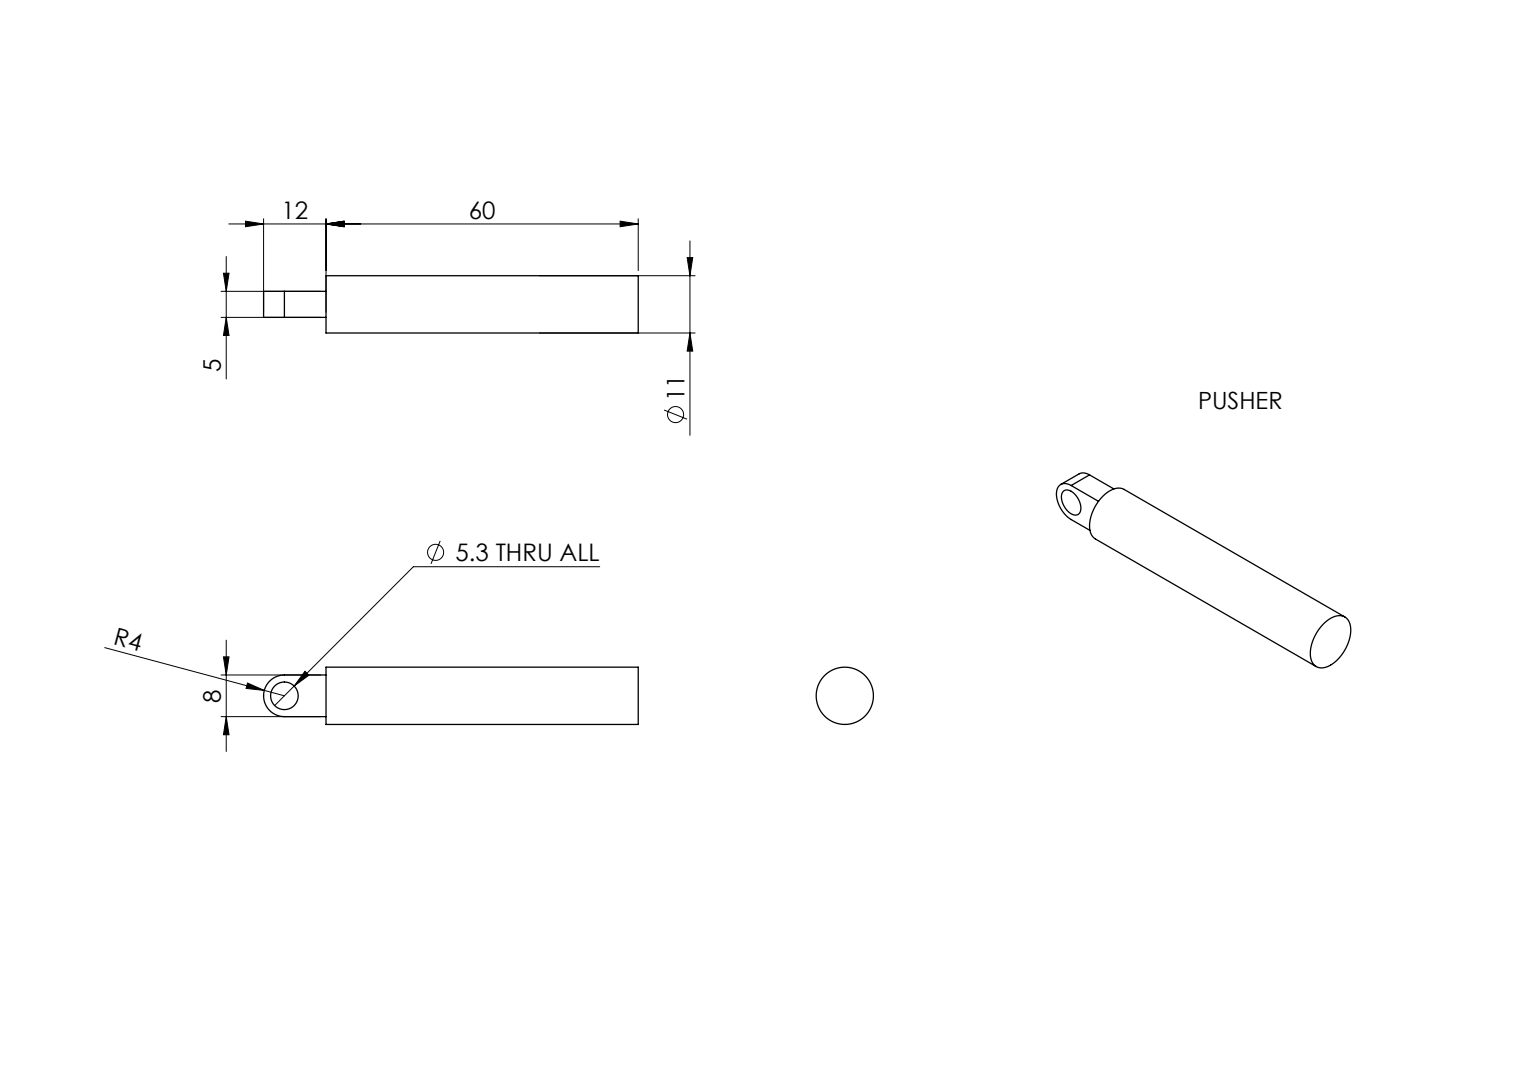
ISO-10303-21;
HEADER;
FILE_DESCRIPTION (('STEP AP214'),
    '1' );
FILE_NAME ('pusher.step',
    '2026-10-31T03:36:27',
    ( '' ),
    ( '' ),
    'SwSTEP 2.0',
    'SolidWorks 2026',
    '' );
FILE_SCHEMA (( 'AUTOMOTIVE_DESIGN' ));
ENDSEC;

DATA;
#89=DIRECTION ( 'NONE',  ( -1.000000000000000000, -6.123233995736766036E-17, 0.000000000000000000 ) ) ;
#381=VECTOR ( 'NONE', #24853, 1000.000000000000000 ) ;
#405=CARTESIAN_POINT ( 'NONE',  ( -69.00000000000002842, 214.0000000000000000, -2.499999999999998668 ) ) ;
#724=AXIS2_PLACEMENT_3D ( 'NONE', #30085, #15119, #33117 ) ;
#815=VERTEX_POINT ( 'NONE', #7521 ) ;
#993=EDGE_LOOP ( 'NONE', ( #26998, #21016, #13480, #17384 ) ) ;
#1044=CARTESIAN_POINT ( 'NONE',  ( -81.00000000000002842, 210.0000000000000000, 2.500000000000001332 ) ) ;
#1193=AXIS2_PLACEMENT_3D ( 'NONE', #20299, #5873, #32024 ) ;
#1362=UNCERTAINTY_MEASURE_WITH_UNIT (LENGTH_MEASURE( 1.000000000000000082E-05 ), #30394, 'distance_accuracy_value', 'NONE');
#1421=ORIENTED_EDGE ( 'NONE', *, *, #25932, .T. ) ;
#1435=DIRECTION ( 'NONE',  ( -1.000000000000000000, -6.123233995736766036E-17, 0.000000000000000000 ) ) ;
#1515=ORIENTED_EDGE ( 'NONE', *, *, #28122, .T. ) ;
#1630=EDGE_CURVE ( 'NONE', #12051, #26056, #3822, .T. ) ;
#1711=CIRCLE ( 'NONE', #36816, 4.000000000000003553 ) ;
#1772=DIRECTION ( 'NONE',  ( 0.000000000000000000, -0.000000000000000000, 1.000000000000000000 ) ) ;
#1802=CARTESIAN_POINT ( 'NONE',  ( -81.00000000000002842, 206.0000000000000000, -2.499999999999998668 ) ) ;
#1831=EDGE_CURVE ( 'NONE', #37491, #32439, #17831, .T. ) ;
#1850=EDGE_LOOP ( 'NONE', ( #28320, #13238, #13654, #30388 ) ) ;
#1911=ORIENTED_EDGE ( 'NONE', *, *, #28122, .F. ) ;
#2035=ORIENTED_EDGE ( 'NONE', *, *, #13992, .T. ) ;
#2126=UNCERTAINTY_MEASURE_WITH_UNIT (LENGTH_MEASURE( 1.000000000000000082E-05 ), #20862, 'distance_accuracy_value', 'NONE');
#2132=PRESENTATION_STYLE_ASSIGNMENT (( #28100 ) ) ;
#2262=VERTEX_POINT ( 'NONE', #29366 ) ;
#2357=VERTEX_POINT ( 'NONE', #405 ) ;
#2450=EDGE_LOOP ( 'NONE', ( #21675, #11995 ) ) ;
#2453=DIRECTION ( 'NONE',  ( -0.000000000000000000, 0.000000000000000000, -1.000000000000000000 ) ) ;
#2550=DIRECTION ( 'NONE',  ( 1.659705900203722642E-32, -2.710505431213758127E-16, -1.000000000000000000 ) ) ;
#2706=CARTESIAN_POINT ( 'NONE',  ( -81.00000000000002842, 206.0000000000000000, 2.500000000000002220 ) ) ;
#2729=CARTESIAN_POINT ( 'NONE',  ( -77.00000000000002842, 210.0000000000000000, -2.499999999999998668 ) ) ;
#2863=EDGE_CURVE ( 'NONE', #23355, #12420, #31331, .T. ) ;
#2931=ORIENTED_EDGE ( 'NONE', *, *, #14124, .T. ) ;
#3005=APPLICATION_CONTEXT ( 'automotive_design' ) ;
#3086=CIRCLE ( 'NONE', #4905, 4.000000000000003553 ) ;
#3101=DIRECTION ( 'NONE',  ( 1.000000000000000000, 6.123233995736766036E-17, -0.000000000000000000 ) ) ;
#3149=CARTESIAN_POINT ( 'NONE',  ( -69.00000000000002842, 210.0000000000000000, 0.000000000000000000 ) ) ;
#3179=ORIENTED_EDGE ( 'NONE', *, *, #27550, .T. ) ;
#3259=CARTESIAN_POINT ( 'NONE',  ( -69.00000000000002842, 206.0000000000000000, 2.500000000000002220 ) ) ;
#3322=ORIENTED_EDGE ( 'NONE', *, *, #16398, .T. ) ;
#3446=ADVANCED_FACE ( 'NONE', ( #16857 ), #11157, .F. ) ;
#3460=CARTESIAN_POINT ( 'NONE',  ( -77.00000000000002842, 206.0000000000000000, 2.500000000000002220 ) ) ;
#3489=FACE_OUTER_BOUND ( 'NONE', #993, .T. ) ;
#3523=EDGE_LOOP ( 'NONE', ( #30051, #36717 ) ) ;
#3627=DIRECTION ( 'NONE',  ( 0.000000000000000000, -1.000000000000000000, 0.000000000000000000 ) ) ;
#3812=EDGE_CURVE ( 'NONE', #27158, #34283, #15876, .T. ) ;
#3822=CIRCLE ( 'NONE', #29851, 2.649999999999999467 ) ;
#3891=AXIS2_PLACEMENT_3D ( 'NONE', #8061, #2550, #6277 ) ;
#4004=DIRECTION ( 'NONE',  ( -0.000000000000000000, -0.000000000000000000, -1.000000000000000000 ) ) ;
#4041=AXIS2_PLACEMENT_3D ( 'NONE', #30951, #17105, #10662 ) ;
#4088=PLANE ( 'NONE',  #11659 ) ;
#4609=DIRECTION ( 'NONE',  ( 1.000000000000000000, 6.123233995736766036E-17, 0.000000000000000000 ) ) ;
#4651=DIRECTION ( 'NONE',  ( 0.000000000000000000, 0.000000000000000000, 1.000000000000000000 ) ) ;
#4762=DIRECTION ( 'NONE',  ( -1.659705900203722642E-32, 2.710505431213758127E-16, 1.000000000000000000 ) ) ;
#4766=ORIENTED_EDGE ( 'NONE', *, *, #18461, .F. ) ;
#4775=CARTESIAN_POINT ( 'NONE',  ( -69.00000000000002842, 206.0000000000000000, -2.499999999999998668 ) ) ;
#4905=AXIS2_PLACEMENT_3D ( 'NONE', #10816, #16142, #10443 ) ;
#4970=CARTESIAN_POINT ( 'NONE',  ( -74.35000000000002274, 210.0000000000000000, 5.000000000000000000 ) ) ;
#4973=SURFACE_STYLE_FILL_AREA ( #36251 ) ;
#4979=PLANE ( 'NONE',  #14973 ) ;
#5010=AXIS2_PLACEMENT_3D ( 'NONE', #7498, #24558, #19074 ) ;
#5293=ORIENTED_EDGE ( 'NONE', *, *, #27550, .F. ) ;
#5521=CYLINDRICAL_SURFACE ( 'NONE', #4041, 5.500000000000005329 ) ;
#5525=CARTESIAN_POINT ( 'NONE',  ( -77.00000000000002842, 214.0000000000000000, -2.499999999999998668 ) ) ;
#5671=CIRCLE ( 'NONE', #6276, 5.500000000000005329 ) ;
#5854=FACE_BOUND ( 'NONE', #17149, .T. ) ;
#5873=DIRECTION ( 'NONE',  ( -1.000000000000000000, -6.123233995736766036E-17, 0.000000000000000000 ) ) ;
#6115=VECTOR ( 'NONE', #25968, 1000.000000000000000 ) ;
#6276=AXIS2_PLACEMENT_3D ( 'NONE', #21708, #24542, #32879 ) ;
#6277=DIRECTION ( 'NONE',  ( 0.000000000000000000, 1.000000000000000000, -3.273063162220408568E-16 ) ) ;
#6300=EDGE_CURVE ( 'NONE', #12051, #34283, #28629, .T. ) ;
#6339=DIRECTION ( 'NONE',  ( -0.000000000000000000, -0.000000000000000000, 1.000000000000000000 ) ) ;
#6347=CARTESIAN_POINT ( 'NONE',  ( -81.00000000000002842, 210.0000000000000000, -2.499999999999998668 ) ) ;
#6359=EDGE_LOOP ( 'NONE', ( #16449, #32660, #37421, #24323 ) ) ;
#6405=EDGE_LOOP ( 'NONE', ( #22858, #25663, #2931, #16829, #11316 ) ) ;
#6528=CARTESIAN_POINT ( 'NONE',  ( -77.00000000000002842, 210.0000000000000000, 5.000000000000000000 ) ) ;
#6534=DIRECTION ( 'NONE',  ( 6.123233995736766036E-17, -1.000000000000000000, 0.000000000000000000 ) ) ;
#6740=DIRECTION ( 'NONE',  ( 0.000000000000000000, 0.000000000000000000, 1.000000000000000000 ) ) ;
#6937=VECTOR ( 'NONE', #24097, 1000.000000000000000 ) ;
#7125=CARTESIAN_POINT ( 'NONE',  ( -77.00000000000002842, 210.0000000000000000, 0.000000000000000000 ) ) ;
#7239=LINE ( 'NONE', #13107, #26015 ) ;
#7292=DIRECTION ( 'NONE',  ( -1.659705900203722642E-32, 2.710505431213758127E-16, 1.000000000000000000 ) ) ;
#7314=DIRECTION ( 'NONE',  ( 1.000000000000000000, 0.000000000000000000, -0.000000000000000000 ) ) ;
#7473=ORIENTED_EDGE ( 'NONE', *, *, #16912, .T. ) ;
#7498=CARTESIAN_POINT ( 'NONE',  ( -9.000000000000024869, 210.0000000000000000, 0.000000000000000000 ) ) ;
#7521=CARTESIAN_POINT ( 'NONE',  ( -77.00000000000002842, 214.0000000000000000, -2.499999999999998668 ) ) ;
#7829=CARTESIAN_POINT ( 'NONE',  ( -81.00000000000002842, 214.0000000000000000, -2.499999999999998668 ) ) ;
#7839=CARTESIAN_POINT ( 'NONE',  ( -81.00000000000002842, 214.0000000000000000, -2.499999999999998668 ) ) ;
#8011=LINE ( 'NONE', #7829, #22826 ) ;
#8061=CARTESIAN_POINT ( 'NONE',  ( -77.00000000000002842, 210.0000000000000000, 2.500000000000001332 ) ) ;
#8248=DIRECTION ( 'NONE',  ( 0.000000000000000000, -0.000000000000000000, 1.000000000000000000 ) ) ;
#8585=DIRECTION ( 'NONE',  ( -1.000000000000000000, -6.123233995736766036E-17, 0.000000000000000000 ) ) ;
#8679=CARTESIAN_POINT ( 'NONE',  ( -77.00000000000002842, 214.0000000000000000, 2.500000000000000000 ) ) ;
#8689=ORIENTED_EDGE ( 'NONE', *, *, #32176, .F. ) ;
#8734=PRODUCT_DEFINITION_FORMATION_WITH_SPECIFIED_SOURCE ( 'ANY', '', #37371, .NOT_KNOWN. ) ;
#8743=DIRECTION ( 'NONE',  ( 1.659705900203722642E-32, -2.710505431213758127E-16, -1.000000000000000000 ) ) ;
#8774=DIRECTION ( 'NONE',  ( -0.000000000000000000, -0.000000000000000000, -1.000000000000000000 ) ) ;
#9133=VECTOR ( 'NONE', #17110, 1000.000000000000000 ) ;
#9159=ORIENTED_EDGE ( 'NONE', *, *, #37039, .F. ) ;
#9224=LINE ( 'NONE', #20990, #13139 ) ;
#9590=AXIS2_PLACEMENT_3D ( 'NONE', #15254, #27183, #6534 ) ;
#9662=( NAMED_UNIT ( * ) PLANE_ANGLE_UNIT ( ) SI_UNIT ( $, .RADIAN. ) );
#9682=ORIENTED_EDGE ( 'NONE', *, *, #36803, .T. ) ;
#9903=AXIS2_PLACEMENT_3D ( 'NONE', #7125, #6740, #18315 ) ;
#9929=DIRECTION ( 'NONE',  ( 1.000000000000000000, 0.000000000000000000, 0.000000000000000000 ) ) ;
#10065=EDGE_CURVE ( 'NONE', #2262, #12420, #12265, .T. ) ;
#10071=EDGE_CURVE ( 'NONE', #2262, #26075, #34298, .T. ) ;
#10173=FACE_OUTER_BOUND ( 'NONE', #6359, .T. ) ;
#10277=ADVANCED_FACE ( 'NONE', ( #5854, #31452 ), #4088, .F. ) ;
#10304=VECTOR ( 'NONE', #30574, 1000.000000000000000 ) ;
#10325=EDGE_CURVE ( 'NONE', #21823, #14348, #30432, .T. ) ;
#10430=DIRECTION ( 'NONE',  ( 1.000000000000000000, 6.123233995736766036E-17, -0.000000000000000000 ) ) ;
#10443=DIRECTION ( 'NONE',  ( 1.000000000000000000, 0.000000000000000000, 0.000000000000000000 ) ) ;
#10487=DIRECTION ( 'NONE',  ( 1.000000000000000000, 0.000000000000000000, 0.000000000000000000 ) ) ;
#10662=DIRECTION ( 'NONE',  ( 0.000000000000000000, -1.000000000000000000, 0.000000000000000000 ) ) ;
#10816=CARTESIAN_POINT ( 'NONE',  ( -77.00000000000002842, 210.0000000000000000, -2.499999999999998668 ) ) ;
#10849=FACE_OUTER_BOUND ( 'NONE', #16526, .T. ) ;
#10916=FACE_OUTER_BOUND ( 'NONE', #18657, .T. ) ;
#10984=ORIENTED_EDGE ( 'NONE', *, *, #10071, .T. ) ;
#11076=AXIS2_PLACEMENT_3D ( 'NONE', #33553, #2453, #16876 ) ;
#11092=STYLED_ITEM ( 'NONE', ( #2132 ), #27327 ) ;
#11157=CYLINDRICAL_SURFACE ( 'NONE', #22531, 2.649999999999999467 ) ;
#11316=ORIENTED_EDGE ( 'NONE', *, *, #25932, .F. ) ;
#11384=CARTESIAN_POINT ( 'NONE',  ( -74.35000000000002274, 210.0000000000000000, -2.499999999999998668 ) ) ;
#11530=VERTEX_POINT ( 'NONE', #8679 ) ;
#11574=DIRECTION ( 'NONE',  ( -0.000000000000000000, -0.000000000000000000, 1.000000000000000000 ) ) ;
#11609=CARTESIAN_POINT ( 'NONE',  ( -81.00000000000002842, 206.0000000000000000, -2.499999999999998668 ) ) ;
#11659=AXIS2_PLACEMENT_3D ( 'NONE', #1802, #30245, #7314 ) ;
#11676=ADVANCED_FACE ( 'NONE', ( #10173 ), #29889, .T. ) ;
#11984=LINE ( 'NONE', #29224, #22400 ) ;
#11995=ORIENTED_EDGE ( 'NONE', *, *, #32176, .T. ) ;
#12051=VERTEX_POINT ( 'NONE', #25137 ) ;
#12152=DIRECTION ( 'NONE',  ( -1.000000000000000000, -6.123233995736766036E-17, 0.000000000000000000 ) ) ;
#12216=ADVANCED_FACE ( 'NONE', ( #10916 ), #34039, .T. ) ;
#12265=CIRCLE ( 'NONE', #11076, 4.000000000000003553 ) ;
#12420=VERTEX_POINT ( 'NONE', #6347 ) ;
#12453=ADVANCED_FACE ( 'NONE', ( #30408, #33247 ), #15631, .T. ) ;
#12533=LINE ( 'NONE', #35453, #6937 ) ;
#12549=CARTESIAN_POINT ( 'NONE',  ( -74.35000000000002274, 210.0000000000000000, 2.500000000000001332 ) ) ;
#12693=APPLICATION_CONTEXT ( 'automotive_design' ) ;
#12839=EDGE_CURVE ( 'NONE', #11530, #23355, #1711, .T. ) ;
#13107=CARTESIAN_POINT ( 'NONE',  ( -77.00000000000002842, 206.0000000000000000, -2.499999999999998668 ) ) ;
#13139=VECTOR ( 'NONE', #1435, 1000.000000000000000 ) ;
#13238=ORIENTED_EDGE ( 'NONE', *, *, #25674, .F. ) ;
#13329=SURFACE_SIDE_STYLE ('',( #4973 ) ) ;
#13480=ORIENTED_EDGE ( 'NONE', *, *, #3812, .F. ) ;
#13510=DIRECTION ( 'NONE',  ( -0.000000000000000000, -0.000000000000000000, 1.000000000000000000 ) ) ;
#13654=ORIENTED_EDGE ( 'NONE', *, *, #28096, .T. ) ;
#13710=( LENGTH_UNIT ( ) NAMED_UNIT ( * ) SI_UNIT ( .MILLI., .METRE. ) );
#13868=CARTESIAN_POINT ( 'NONE',  ( -69.00000000000002842, 206.0000000000000000, -2.499999999999998668 ) ) ;
#13930=ORIENTED_EDGE ( 'NONE', *, *, #25674, .T. ) ;
#13992=EDGE_CURVE ( 'NONE', #14430, #2262, #7239, .T. ) ;
#14004=DIRECTION ( 'NONE',  ( -0.000000000000000000, -0.000000000000000000, 1.000000000000000000 ) ) ;
#14124=EDGE_CURVE ( 'NONE', #14430, #37491, #31894, .T. ) ;
#14260=AXIS2_PLACEMENT_3D ( 'NONE', #2729, #8248, #37224 ) ;
#14326=VECTOR ( 'NONE', #13510, 1000.000000000000000 ) ;
#14348=VERTEX_POINT ( 'NONE', #24321 ) ;
#14430=VERTEX_POINT ( 'NONE', #3460 ) ;
#14481=ORIENTED_EDGE ( 'NONE', *, *, #1630, .T. ) ;
#14680=EDGE_CURVE ( 'NONE', #26075, #37491, #19393, .T. ) ;
#14719=COLOUR_RGB ( '',0.8941176470588234615, 0.8941176470588234615, 0.8941176470588234615 ) ;
#14973=AXIS2_PLACEMENT_3D ( 'NONE', #7839, #25266, #4609 ) ;
#15119=DIRECTION ( 'NONE',  ( 1.659705900203722642E-32, -2.710505431213758127E-16, -1.000000000000000000 ) ) ;
#15236=CARTESIAN_POINT ( 'NONE',  ( -81.00000000000002842, 214.0000000000000000, 2.500000000000000000 ) ) ;
#15254=CARTESIAN_POINT ( 'NONE',  ( -69.00000000000002842, 210.0000000000000000, 0.000000000000000000 ) ) ;
#15631=PLANE ( 'NONE',  #9590 ) ;
#15748=AXIS2_PLACEMENT_3D ( 'NONE', #11609, #20347, #8585 ) ;
#15876=CIRCLE ( 'NONE', #724, 2.649999999999985700 ) ;
#15940=ORIENTED_EDGE ( 'NONE', *, *, #25175, .F. ) ;
#15949=MECHANICAL_DESIGN_GEOMETRIC_PRESENTATION_REPRESENTATION('',(#11092),#31695);
#16017=DIRECTION ( 'NONE',  ( 0.000000000000000000, 1.000000000000000000, -2.168404344971006896E-16 ) ) ;
#16047=CARTESIAN_POINT ( 'NONE',  ( 0.000000000000000000, 0.000000000000000000, 0.000000000000000000 ) ) ;
#16052=SHAPE_DEFINITION_REPRESENTATION ( #22565, #35512 ) ;
#16061=CARTESIAN_POINT ( 'NONE',  ( -77.00000000000002842, 210.0000000000000000, 0.000000000000000000 ) ) ;
#16142=DIRECTION ( 'NONE',  ( -0.000000000000000000, 0.000000000000000000, -1.000000000000000000 ) ) ;
#16148=ORIENTED_EDGE ( 'NONE', *, *, #29038, .T. ) ;
#16339=EDGE_LOOP ( 'NONE', ( #29976, #36526, #5293, #16687 ) ) ;
#16398=EDGE_CURVE ( 'NONE', #815, #11530, #23730, .T. ) ;
#16449=ORIENTED_EDGE ( 'NONE', *, *, #16398, .F. ) ;
#16526=EDGE_LOOP ( 'NONE', ( #9159, #18884, #16148, #8689 ) ) ;
#16687=ORIENTED_EDGE ( 'NONE', *, *, #19704, .F. ) ;
#16711=DIRECTION ( 'NONE',  ( 0.000000000000000000, 1.000000000000000000, -2.168404344971006896E-16 ) ) ;
#16829=ORIENTED_EDGE ( 'NONE', *, *, #1831, .T. ) ;
#16851=AXIS2_PLACEMENT_3D ( 'NONE', #26426, #89, #37425 ) ;
#16857=FACE_OUTER_BOUND ( 'NONE', #1850, .T. ) ;
#16876=DIRECTION ( 'NONE',  ( 1.000000000000000000, 0.000000000000000000, 0.000000000000000000 ) ) ;
#16912=EDGE_CURVE ( 'NONE', #12420, #815, #3086, .T. ) ;
#17105=DIRECTION ( 'NONE',  ( -1.000000000000000000, -6.123233995736766036E-17, 0.000000000000000000 ) ) ;
#17110=DIRECTION ( 'NONE',  ( -0.000000000000000000, -0.000000000000000000, 1.000000000000000000 ) ) ;
#17149=EDGE_LOOP ( 'NONE', ( #13930, #14481 ) ) ;
#17215=AXIS2_PLACEMENT_3D ( 'NONE', #16047, #4651, #19645 ) ;
#17384=ORIENTED_EDGE ( 'NONE', *, *, #28096, .F. ) ;
#17568=ORIENTED_EDGE ( 'NONE', *, *, #37039, .T. ) ;
#17831=LINE ( 'NONE', #3259, #6115 ) ;
#18063=CLOSED_SHELL ( 'NONE', ( #30103, #12216, #28031, #18693, #12453, #20499, #30224, #10277, #19793, #11676, #32555, #3446 ) ) ;
#18315=DIRECTION ( 'NONE',  ( 1.000000000000000000, 0.000000000000000000, 0.000000000000000000 ) ) ;
#18461=EDGE_CURVE ( 'NONE', #23355, #14430, #30895, .T. ) ;
#18630=CARTESIAN_POINT ( 'NONE',  ( -69.00000000000002842, 206.0000000000000000, -2.499999999999998668 ) ) ;
#18657=EDGE_LOOP ( 'NONE', ( #26819, #17568, #15940, #25194 ) ) ;
#18693=ADVANCED_FACE ( 'NONE', ( #34501 ), #34681, .F. ) ;
#18884=ORIENTED_EDGE ( 'NONE', *, *, #10325, .T. ) ;
#18898=CARTESIAN_POINT ( 'NONE',  ( -9.000000000000024869, 210.0000000000000000, 0.000000000000000000 ) ) ;
#18959=DIRECTION ( 'NONE',  ( 1.000000000000000000, 0.000000000000000000, 0.000000000000000000 ) ) ;
#19035=( NAMED_UNIT ( * ) SI_UNIT ( $, .STERADIAN. ) SOLID_ANGLE_UNIT ( ) );
#19074=DIRECTION ( 'NONE',  ( 0.000000000000000000, -1.000000000000000000, 0.000000000000000000 ) ) ;
#19384=AXIS2_PLACEMENT_3D ( 'NONE', #22583, #4762, #16711 ) ;
#19393=LINE ( 'NONE', #4775, #10304 ) ;
#19645=DIRECTION ( 'NONE',  ( 1.000000000000000000, 0.000000000000000000, 0.000000000000000000 ) ) ;
#19704=EDGE_CURVE ( 'NONE', #32439, #2357, #11984, .T. ) ;
#19793=ADVANCED_FACE ( 'NONE', ( #20716 ), #35283, .F. ) ;
#20086=ORIENTED_EDGE ( 'NONE', *, *, #14124, .F. ) ;
#20161=DIRECTION ( 'NONE',  ( 1.000000000000000000, 6.123233995736766036E-17, -0.000000000000000000 ) ) ;
#20299=CARTESIAN_POINT ( 'NONE',  ( -9.000000000000024869, 210.0000000000000000, 0.000000000000000000 ) ) ;
#20347=DIRECTION ( 'NONE',  ( -6.123233995736766036E-17, 1.000000000000000000, 0.000000000000000000 ) ) ;
#20499=ADVANCED_FACE ( 'NONE', ( #32040, #31855 ), #23154, .F. ) ;
#20661=MANIFOLD_SOLID_BREP ( 'M5 Clearance Hole1', #18063 ) ;
#20668=( NAMED_UNIT ( * ) SI_UNIT ( $, .STERADIAN. ) SOLID_ANGLE_UNIT ( ) );
#20716=FACE_OUTER_BOUND ( 'NONE', #31605, .T. ) ;
#20862=( LENGTH_UNIT ( ) NAMED_UNIT ( * ) SI_UNIT ( .MILLI., .METRE. ) );
#20990=CARTESIAN_POINT ( 'NONE',  ( -9.000000000000024869, 204.5000000000000000, 0.000000000000000000 ) ) ;
#21016=ORIENTED_EDGE ( 'NONE', *, *, #6300, .T. ) ;
#21127=AXIS2_PLACEMENT_3D ( 'NONE', #16061, #24026, #21565 ) ;
#21247=MECHANICAL_DESIGN_GEOMETRIC_PRESENTATION_REPRESENTATION('',(#26656),#26062);
#21498=ORIENTED_EDGE ( 'NONE', *, *, #14680, .T. ) ;
#21565=DIRECTION ( 'NONE',  ( -1.000000000000000000, 0.000000000000000000, 0.000000000000000000 ) ) ;
#21675=ORIENTED_EDGE ( 'NONE', *, *, #25175, .T. ) ;
#21708=CARTESIAN_POINT ( 'NONE',  ( -69.00000000000002842, 210.0000000000000000, 0.000000000000000000 ) ) ;
#21717=FACE_OUTER_BOUND ( 'NONE', #29264, .T. ) ;
#21823=VERTEX_POINT ( 'NONE', #27063 ) ;
#21836=AXIS2_PLACEMENT_3D ( 'NONE', #34696, #8743, #32231 ) ;
#22071=ORIENTED_EDGE ( 'NONE', *, *, #2863, .T. ) ;
#22373=EDGE_LOOP ( 'NONE', ( #22772, #30540, #7473, #1515, #3179 ) ) ;
#22400=VECTOR ( 'NONE', #8774, 1000.000000000000000 ) ;
#22422=LINE ( 'NONE', #4970, #14326 ) ;
#22426=FILL_AREA_STYLE_COLOUR ( '', #14719 ) ;
#22531=AXIS2_PLACEMENT_3D ( 'NONE', #36742, #14004, #18959 ) ;
#22565=PRODUCT_DEFINITION_SHAPE ( 'NONE', 'NONE',  #29920 ) ;
#22583=CARTESIAN_POINT ( 'NONE',  ( -77.00000000000002842, 210.0000000000000000, 2.500000000000001332 ) ) ;
#22609=DIRECTION ( 'NONE',  ( 1.000000000000000000, 6.123233995736766036E-17, -0.000000000000000000 ) ) ;
#22772=ORIENTED_EDGE ( 'NONE', *, *, #10071, .F. ) ;
#22826=VECTOR ( 'NONE', #22609, 1000.000000000000000 ) ;
#22858=ORIENTED_EDGE ( 'NONE', *, *, #12839, .T. ) ;
#23154=PLANE ( 'NONE',  #21836 ) ;
#23254=ORIENTED_EDGE ( 'NONE', *, *, #10065, .F. ) ;
#23355=VERTEX_POINT ( 'NONE', #1044 ) ;
#23513=EDGE_LOOP ( 'NONE', ( #1911, #3322, #1421, #35854 ) ) ;
#23730=LINE ( 'NONE', #5525, #9133 ) ;
#23971=CYLINDRICAL_SURFACE ( 'NONE', #36749, 2.649999999999999467 ) ;
#24026=DIRECTION ( 'NONE',  ( 0.000000000000000000, 0.000000000000000000, -1.000000000000000000 ) ) ;
#24097=DIRECTION ( 'NONE',  ( -1.000000000000000000, -6.123233995736766036E-17, 0.000000000000000000 ) ) ;
#24321=CARTESIAN_POINT ( 'NONE',  ( -9.000000000000024869, 204.5000000000000000, 0.000000000000000000 ) ) ;
#24323=ORIENTED_EDGE ( 'NONE', *, *, #12839, .F. ) ;
#24542=DIRECTION ( 'NONE',  ( -1.000000000000000000, -6.123233995736766036E-17, 0.000000000000000000 ) ) ;
#24558=DIRECTION ( 'NONE',  ( -1.000000000000000000, -6.123233995736766036E-17, 0.000000000000000000 ) ) ;
#24571=AXIS2_PLACEMENT_3D ( 'NONE', #3149, #26266, #32332 ) ;
#24709=CARTESIAN_POINT ( 'NONE',  ( -77.00000000000002842, 210.0000000000000000, -2.499999999999998668 ) ) ;
#24831=CARTESIAN_POINT ( 'NONE',  ( -81.00000000000002842, 206.0000000000000000, -2.499999999999998668 ) ) ;
#24853=DIRECTION ( 'NONE',  ( -0.000000000000000000, -1.000000000000000000, -0.000000000000000000 ) ) ;
#24887=( NAMED_UNIT ( * ) SI_UNIT ( $, .STERADIAN. ) SOLID_ANGLE_UNIT ( ) );
#25137=CARTESIAN_POINT ( 'NONE',  ( -79.65000000000001990, 210.0000000000000000, -2.499999999999998668 ) ) ;
#25169=CIRCLE ( 'NONE', #24571, 5.500000000000005329 ) ;
#25175=EDGE_CURVE ( 'NONE', #33950, #31726, #25169, .T. ) ;
#25194=ORIENTED_EDGE ( 'NONE', *, *, #29038, .F. ) ;
#25266=DIRECTION ( 'NONE',  ( 6.123233995736766036E-17, -1.000000000000000000, 0.000000000000000000 ) ) ;
#25663=ORIENTED_EDGE ( 'NONE', *, *, #18461, .T. ) ;
#25674=EDGE_CURVE ( 'NONE', #26056, #12051, #36061, .T. ) ;
#25841=CIRCLE ( 'NONE', #32524, 5.500000000000005329 ) ;
#25932=EDGE_CURVE ( 'NONE', #11530, #32439, #29058, .T. ) ;
#25968=DIRECTION ( 'NONE',  ( 0.000000000000000000, 1.000000000000000000, -2.710505431213758620E-16 ) ) ;
#25979=CARTESIAN_POINT ( 'NONE',  ( -79.65000000000001990, 210.0000000000000000, 2.500000000000001332 ) ) ;
#26015=VECTOR ( 'NONE', #4004, 1000.000000000000000 ) ;
#26056=VERTEX_POINT ( 'NONE', #11384 ) ;
#26062=( GEOMETRIC_REPRESENTATION_CONTEXT ( 3 ) GLOBAL_UNCERTAINTY_ASSIGNED_CONTEXT ( ( #2126 ) ) GLOBAL_UNIT_ASSIGNED_CONTEXT ( ( #20862, #9662, #20668 ) ) REPRESENTATION_CONTEXT ( 'NONE', 'WORKASPACE' ) );
#26075=VERTEX_POINT ( 'NONE', #13868 ) ;
#26266=DIRECTION ( 'NONE',  ( -1.000000000000000000, -6.123233995736766036E-17, 0.000000000000000000 ) ) ;
#26426=CARTESIAN_POINT ( 'NONE',  ( -9.000000000000024869, 210.0000000000000000, 0.000000000000000000 ) ) ;
#26526=CARTESIAN_POINT ( 'NONE',  ( -81.00000000000002842, 210.0000000000000000, 0.000000000000000000 ) ) ;
#26656=STYLED_ITEM('',(#37535),#20661);
#26819=ORIENTED_EDGE ( 'NONE', *, *, #29509, .T. ) ;
#26998=ORIENTED_EDGE ( 'NONE', *, *, #1630, .F. ) ;
#27063=CARTESIAN_POINT ( 'NONE',  ( -9.000000000000024869, 215.5000000000000000, 6.735557395310435121E-16 ) ) ;
#27158=VERTEX_POINT ( 'NONE', #12549 ) ;
#27183=DIRECTION ( 'NONE',  ( -1.000000000000000000, -6.123233995736766036E-17, 0.000000000000000000 ) ) ;
#27327=ADVANCED_BREP_SHAPE_REPRESENTATION ( '', ( #20661, #17215 ), #27435 ) ;
#27435=( GEOMETRIC_REPRESENTATION_CONTEXT ( 3 ) GLOBAL_UNCERTAINTY_ASSIGNED_CONTEXT ( ( #1362 ) ) GLOBAL_UNIT_ASSIGNED_CONTEXT ( ( #30394, #33235, #19035 ) ) REPRESENTATION_CONTEXT ( 'NONE', 'WORKASPACE' ) );
#27515=LINE ( 'NONE', #18630, #381 ) ;
#27550=EDGE_CURVE ( 'NONE', #2357, #26075, #27515, .T. ) ;
#28031=ADVANCED_FACE ( 'NONE', ( #10849 ), #5521, .T. ) ;
#28096=EDGE_CURVE ( 'NONE', #26056, #27158, #22422, .T. ) ;
#28100=SURFACE_STYLE_USAGE ( .BOTH. , #13329 ) ;
#28122=EDGE_CURVE ( 'NONE', #815, #2357, #8011, .T. ) ;
#28320=ORIENTED_EDGE ( 'NONE', *, *, #6300, .F. ) ;
#28332=CARTESIAN_POINT ( 'NONE',  ( -69.00000000000002842, 206.0000000000000000, 2.500000000000002220 ) ) ;
#28629=LINE ( 'NONE', #37340, #36054 ) ;
#29038=EDGE_CURVE ( 'NONE', #14348, #33950, #9224, .T. ) ;
#29058=LINE ( 'NONE', #15236, #33631 ) ;
#29224=CARTESIAN_POINT ( 'NONE',  ( -69.00000000000002842, 214.0000000000000000, -2.499999999999998668 ) ) ;
#29264=EDGE_LOOP ( 'NONE', ( #23254, #32180, #4766, #22071 ) ) ;
#29366=CARTESIAN_POINT ( 'NONE',  ( -77.00000000000002842, 206.0000000000000000, -2.499999999999998668 ) ) ;
#29509=EDGE_CURVE ( 'NONE', #14348, #21823, #25841, .T. ) ;
#29851=AXIS2_PLACEMENT_3D ( 'NONE', #24709, #1772, #10487 ) ;
#29889=CYLINDRICAL_SURFACE ( 'NONE', #21127, 4.000000000000003553 ) ;
#29920=PRODUCT_DEFINITION ( 'UNKNOWN', '', #8734, #31963 ) ;
#29976=ORIENTED_EDGE ( 'NONE', *, *, #1831, .F. ) ;
#30051=ORIENTED_EDGE ( 'NONE', *, *, #29509, .F. ) ;
#30085=CARTESIAN_POINT ( 'NONE',  ( -77.00000000000002842, 210.0000000000000000, 2.500000000000001332 ) ) ;
#30103=ADVANCED_FACE ( 'NONE', ( #3489 ), #23971, .F. ) ;
#30224=ADVANCED_FACE ( 'NONE', ( #30773 ), #4979, .F. ) ;
#30245=DIRECTION ( 'NONE',  ( 0.000000000000000000, -0.000000000000000000, 1.000000000000000000 ) ) ;
#30261=PRODUCT_CONTEXT ( 'NONE', #3005, 'mechanical' ) ;
#30388=ORIENTED_EDGE ( 'NONE', *, *, #36803, .F. ) ;
#30394=( LENGTH_UNIT ( ) NAMED_UNIT ( * ) SI_UNIT ( .MILLI., .METRE. ) );
#30408=FACE_BOUND ( 'NONE', #16339, .T. ) ;
#30432=CIRCLE ( 'NONE', #5010, 5.500000000000005329 ) ;
#30540=ORIENTED_EDGE ( 'NONE', *, *, #10065, .T. ) ;
#30574=DIRECTION ( 'NONE',  ( 0.000000000000000000, 0.000000000000000000, 1.000000000000000000 ) ) ;
#30773=FACE_OUTER_BOUND ( 'NONE', #23513, .T. ) ;
#30895=CIRCLE ( 'NONE', #19384, 4.000000000000003553 ) ;
#30951=CARTESIAN_POINT ( 'NONE',  ( -9.000000000000024869, 210.0000000000000000, 0.000000000000000000 ) ) ;
#31302=CARTESIAN_POINT ( 'NONE',  ( -69.00000000000002842, 204.5000000000000000, 0.000000000000000000 ) ) ;
#31331=LINE ( 'NONE', #26526, #31889 ) ;
#31395=CARTESIAN_POINT ( 'NONE',  ( -69.00000000000002842, 215.5000000000000000, 6.735557395310435121E-16 ) ) ;
#31450=EDGE_LOOP ( 'NONE', ( #32460, #9682 ) ) ;
#31452=FACE_OUTER_BOUND ( 'NONE', #22373, .T. ) ;
#31605=EDGE_LOOP ( 'NONE', ( #20086, #2035, #10984, #21498 ) ) ;
#31695=( GEOMETRIC_REPRESENTATION_CONTEXT ( 3 ) GLOBAL_UNCERTAINTY_ASSIGNED_CONTEXT ( ( #32824 ) ) GLOBAL_UNIT_ASSIGNED_CONTEXT ( ( #13710, #36811, #24887 ) ) REPRESENTATION_CONTEXT ( 'NONE', 'WORKASPACE' ) );
#31726=VERTEX_POINT ( 'NONE', #31395 ) ;
#31733=CIRCLE ( 'NONE', #3891, 2.649999999999985700 ) ;
#31855=FACE_OUTER_BOUND ( 'NONE', #6405, .T. ) ;
#31889=VECTOR ( 'NONE', #32405, 1000.000000000000000 ) ;
#31894=LINE ( 'NONE', #2706, #32076 ) ;
#31963=PRODUCT_DEFINITION_CONTEXT ( 'detailed design', #12693, 'design' ) ;
#32024=DIRECTION ( 'NONE',  ( 6.123233995736766036E-17, -1.000000000000000000, 0.000000000000000000 ) ) ;
#32040=FACE_BOUND ( 'NONE', #31450, .T. ) ;
#32076=VECTOR ( 'NONE', #20161, 1000.000000000000000 ) ;
#32176=EDGE_CURVE ( 'NONE', #31726, #33950, #5671, .T. ) ;
#32180=ORIENTED_EDGE ( 'NONE', *, *, #13992, .F. ) ;
#32231=DIRECTION ( 'NONE',  ( 0.000000000000000000, 1.000000000000000000, -2.710505431213758127E-16 ) ) ;
#32332=DIRECTION ( 'NONE',  ( 0.000000000000000000, -1.000000000000000000, 0.000000000000000000 ) ) ;
#32405=DIRECTION ( 'NONE',  ( 0.000000000000000000, 0.000000000000000000, -1.000000000000000000 ) ) ;
#32439=VERTEX_POINT ( 'NONE', #36282 ) ;
#32460=ORIENTED_EDGE ( 'NONE', *, *, #3812, .T. ) ;
#32524=AXIS2_PLACEMENT_3D ( 'NONE', #18898, #12152, #3627 ) ;
#32555=ADVANCED_FACE ( 'NONE', ( #21717 ), #33082, .T. ) ;
#32660=ORIENTED_EDGE ( 'NONE', *, *, #16912, .F. ) ;
#32824=UNCERTAINTY_MEASURE_WITH_UNIT (LENGTH_MEASURE( 1.000000000000000082E-05 ), #13710, 'distance_accuracy_value', 'NONE');
#32874=CARTESIAN_POINT ( 'NONE',  ( -77.00000000000002842, 210.0000000000000000, 2.500000000000001332 ) ) ;
#32879=DIRECTION ( 'NONE',  ( 0.000000000000000000, -1.000000000000000000, 0.000000000000000000 ) ) ;
#33082=CYLINDRICAL_SURFACE ( 'NONE', #9903, 4.000000000000003553 ) ;
#33117=DIRECTION ( 'NONE',  ( 0.000000000000000000, 1.000000000000000000, -3.273063162220408568E-16 ) ) ;
#33235=( NAMED_UNIT ( * ) PLANE_ANGLE_UNIT ( ) SI_UNIT ( $, .RADIAN. ) );
#33247=FACE_OUTER_BOUND ( 'NONE', #2450, .T. ) ;
#33553=CARTESIAN_POINT ( 'NONE',  ( -77.00000000000002842, 210.0000000000000000, -2.499999999999998668 ) ) ;
#33631=VECTOR ( 'NONE', #3101, 1000.000000000000000 ) ;
#33950=VERTEX_POINT ( 'NONE', #31302 ) ;
#34039=CYLINDRICAL_SURFACE ( 'NONE', #16851, 5.500000000000005329 ) ;
#34283=VERTEX_POINT ( 'NONE', #25979 ) ;
#34298=LINE ( 'NONE', #24831, #37095 ) ;
#34501=FACE_OUTER_BOUND ( 'NONE', #3523, .T. ) ;
#34681=PLANE ( 'NONE',  #1193 ) ;
#34696=CARTESIAN_POINT ( 'NONE',  ( -81.00000000000002842, 206.0000000000000000, 2.500000000000002220 ) ) ;
#35283=PLANE ( 'NONE',  #15748 ) ;
#35453=CARTESIAN_POINT ( 'NONE',  ( -9.000000000000024869, 215.5000000000000000, 6.735557395310442023E-16 ) ) ;
#35512=SHAPE_REPRESENTATION ( 'pusher', ( #17215 ), #27435 ) ;
#35854=ORIENTED_EDGE ( 'NONE', *, *, #19704, .T. ) ;
#36054=VECTOR ( 'NONE', #11574, 1000.000000000000000 ) ;
#36061=CIRCLE ( 'NONE', #14260, 2.649999999999999467 ) ;
#36251=FILL_AREA_STYLE ('',( #22426 ) ) ;
#36282=CARTESIAN_POINT ( 'NONE',  ( -69.00000000000002842, 214.0000000000000000, 2.500000000000000000 ) ) ;
#36435=SHAPE_REPRESENTATION_RELATIONSHIP ( 'NONE' , 'NONE' ,  #35512, #27327 ) ;
#36526=ORIENTED_EDGE ( 'NONE', *, *, #14680, .F. ) ;
#36717=ORIENTED_EDGE ( 'NONE', *, *, #10325, .F. ) ;
#36742=CARTESIAN_POINT ( 'NONE',  ( -77.00000000000002842, 210.0000000000000000, 5.000000000000000000 ) ) ;
#36749=AXIS2_PLACEMENT_3D ( 'NONE', #6528, #6339, #9929 ) ;
#36803=EDGE_CURVE ( 'NONE', #34283, #27158, #31733, .T. ) ;
#36811=( NAMED_UNIT ( * ) PLANE_ANGLE_UNIT ( ) SI_UNIT ( $, .RADIAN. ) );
#36816=AXIS2_PLACEMENT_3D ( 'NONE', #32874, #7292, #16017 ) ;
#37039=EDGE_CURVE ( 'NONE', #21823, #31726, #12533, .T. ) ;
#37095=VECTOR ( 'NONE', #10430, 1000.000000000000000 ) ;
#37224=DIRECTION ( 'NONE',  ( 1.000000000000000000, 0.000000000000000000, 0.000000000000000000 ) ) ;
#37340=CARTESIAN_POINT ( 'NONE',  ( -79.65000000000001990, 210.0000000000000000, 5.000000000000000000 ) ) ;
#37371=PRODUCT ( 'pusher', 'pusher', '', ( #30261 ) ) ;
#37421=ORIENTED_EDGE ( 'NONE', *, *, #2863, .F. ) ;
#37425=DIRECTION ( 'NONE',  ( 0.000000000000000000, -1.000000000000000000, 0.000000000000000000 ) ) ;
#37491=VERTEX_POINT ( 'NONE', #28332 ) ;
#37529=COLOUR_RGB('Sky Blue',0.24,0.69,0.87);
#37530=FILL_AREA_STYLE_COLOUR('',#37529);
#37531=FILL_AREA_STYLE('',(#37530));
#37532=SURFACE_STYLE_FILL_AREA(#37531);
#37533=SURFACE_SIDE_STYLE('',(#37532));
#37534=SURFACE_STYLE_USAGE(.BOTH.,#37533);
#37535=PRESENTATION_STYLE_ASSIGNMENT((#37534));
ENDSEC;
END-ISO-10303-21;
